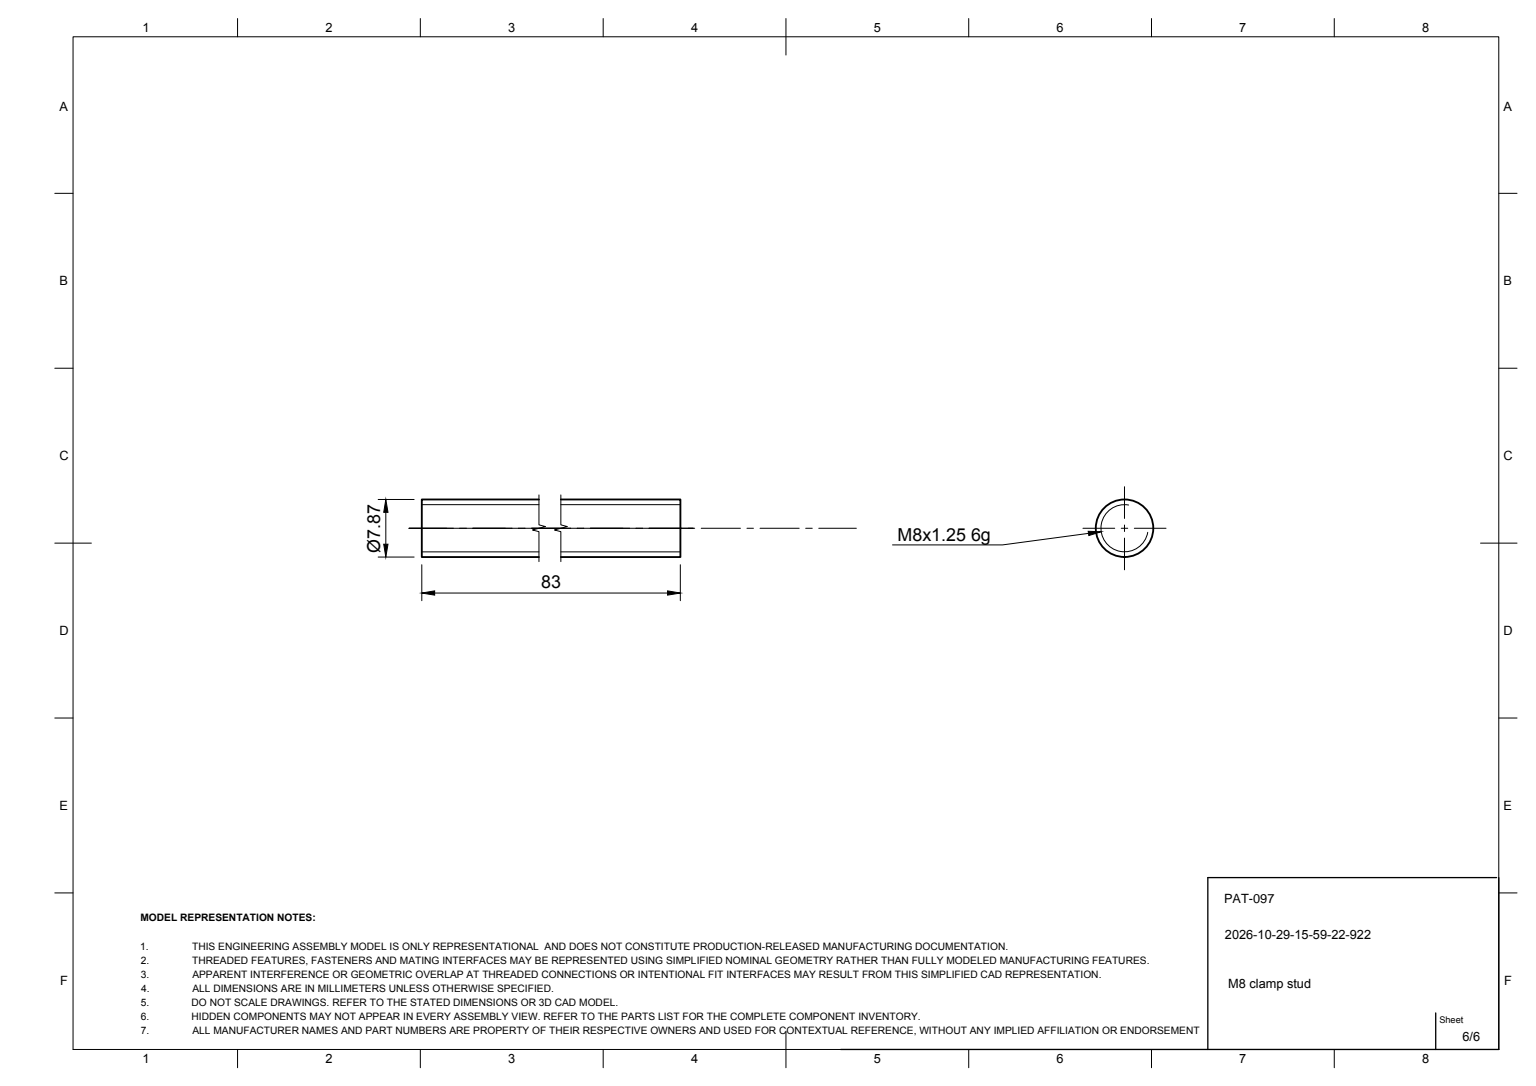
ISO-10303-21;
HEADER;
/* Generated by software containing ST-Developer
 * from STEP Tools, Inc. (www.steptools.com) 
 */

FILE_DESCRIPTION(
/* description */ ('PAT-097'),
/* implementation_level */ '2;1');

FILE_NAME(
/* name */ 'M8 clamp stud.step',
/* time_stamp */ '2026-10-29T15:59:31-07:00',
/* author */ (''),
/* organization */ (''),
/* preprocessor_version */ 'ST-DEVELOPER v20.2',
/* originating_system */ 'Autodesk Translation Framework v15.17.0.0',
/* authorisation */ '');

FILE_SCHEMA (('AUTOMOTIVE_DESIGN { 1 0 10303 214 3 1 1 }'));
ENDSEC;

DATA;
#10=MECHANICAL_DESIGN_GEOMETRIC_PRESENTATION_REPRESENTATION('',(#79),#2768);
#65=SHAPE_REPRESENTATION_RELATIONSHIP('SRR','None',#2803,#72);
#72=ADVANCED_BREP_SHAPE_REPRESENTATION('',(#86),#2765);
#79=STYLED_ITEM('',(#2918),#86);
#86=MANIFOLD_SOLID_BREP('Body1',#1600);
#112=CYLINDRICAL_SURFACE('',#1798,0.3933);
#210=CIRCLE('',#1799,0.3933);
#211=CIRCLE('',#1800,0.3933);
#285=FACE_OUTER_BOUND('',#412,.T.);
#286=FACE_OUTER_BOUND('',#413,.T.);
#287=FACE_OUTER_BOUND('',#414,.T.);
#412=EDGE_LOOP('',(#1391,#1392,#1393,#1394));
#413=EDGE_LOOP('',(#1395));
#414=EDGE_LOOP('',(#1396));
#559=LINE('',#2646,#696);
#696=VECTOR('',#2200,0.4);
#822=VERTEX_POINT('',#2643);
#823=VERTEX_POINT('',#2645);
#1015=EDGE_CURVE('',#822,#822,#210,.F.);
#1016=EDGE_CURVE('',#822,#823,#559,.T.);
#1017=EDGE_CURVE('',#823,#823,#211,.F.);
#1391=ORIENTED_EDGE('',*,*,#1015,.F.);
#1392=ORIENTED_EDGE('',*,*,#1016,.T.);
#1393=ORIENTED_EDGE('',*,*,#1017,.T.);
#1394=ORIENTED_EDGE('',*,*,#1016,.F.);
#1395=ORIENTED_EDGE('',*,*,#1015,.T.);
#1396=ORIENTED_EDGE('',*,*,#1017,.F.);
#1501=PLANE('',#1801);
#1502=PLANE('',#1802);
#1578=ADVANCED_FACE('',(#285),#112,.T.);
#1579=ADVANCED_FACE('',(#286),#1501,.T.);
#1580=ADVANCED_FACE('',(#287),#1502,.F.);
#1600=CLOSED_SHELL('',(#1578,#1579,#1580));
#1797=AXIS2_PLACEMENT_3D('',#2641,#2194,#2195);
#1798=AXIS2_PLACEMENT_3D('',#2642,#2196,#2197);
#1799=AXIS2_PLACEMENT_3D('',#2644,#2198,#2199);
#1800=AXIS2_PLACEMENT_3D('',#2647,#2201,#2202);
#1801=AXIS2_PLACEMENT_3D('',#2648,#2203,#2204);
#1802=AXIS2_PLACEMENT_3D('',#2649,#2205,#2206);
#2194=DIRECTION('axis',(0.,0.,1.));
#2195=DIRECTION('refdir',(1.,0.,0.));
#2196=DIRECTION('center_axis',(0.,0.,1.));
#2197=DIRECTION('ref_axis',(1.,0.,0.));
#2198=DIRECTION('center_axis',(0.,0.,-1.));
#2199=DIRECTION('ref_axis',(1.,0.,0.));
#2200=DIRECTION('',(0.,0.,-1.));
#2201=DIRECTION('center_axis',(0.,0.,-1.));
#2202=DIRECTION('ref_axis',(1.,0.,0.));
#2203=DIRECTION('center_axis',(0.,0.,1.));
#2204=DIRECTION('ref_axis',(1.,0.,0.));
#2205=DIRECTION('center_axis',(0.,0.,1.));
#2206=DIRECTION('ref_axis',(1.,0.,0.));
#2641=CARTESIAN_POINT('',(0.,0.,0.));
#2642=CARTESIAN_POINT('Origin',(10.,-4.,0.));
#2643=CARTESIAN_POINT('',(9.6067,-4.,8.3));
#2644=CARTESIAN_POINT('Origin',(10.,-4.,8.3));
#2645=CARTESIAN_POINT('',(9.6067,-4.,0.));
#2646=CARTESIAN_POINT('',(9.6067,-4.,0.));
#2647=CARTESIAN_POINT('Origin',(10.,-4.,0.));
#2648=CARTESIAN_POINT('Origin',(10.,-4.,8.3));
#2649=CARTESIAN_POINT('Origin',(10.,-4.,0.));
#2756=UNCERTAINTY_MEASURE_WITH_UNIT(LENGTH_MEASURE(0.001),#2769,
'DISTANCE_ACCURACY_VALUE',
'Maximum model space distance between geometric entities at asserted c
onnectivities');
#2759=UNCERTAINTY_MEASURE_WITH_UNIT(LENGTH_MEASURE(0.001),#2769,
'DISTANCE_ACCURACY_VALUE',
'Maximum model space distance between geometric entities at asserted c
onnectivities');
#2765=(
GEOMETRIC_REPRESENTATION_CONTEXT(3)
GLOBAL_UNCERTAINTY_ASSIGNED_CONTEXT((#2756))
GLOBAL_UNIT_ASSIGNED_CONTEXT((#2769,#2771,#2772))
REPRESENTATION_CONTEXT('','3D')
);
#2768=(
GEOMETRIC_REPRESENTATION_CONTEXT(3)
GLOBAL_UNCERTAINTY_ASSIGNED_CONTEXT((#2759))
GLOBAL_UNIT_ASSIGNED_CONTEXT((#2769,#2771,#2772))
REPRESENTATION_CONTEXT('','3D')
);
#2769=(
LENGTH_UNIT()
NAMED_UNIT(*)
SI_UNIT(.CENTI.,.METRE.)
);
#2771=(
NAMED_UNIT(*)
PLANE_ANGLE_UNIT()
SI_UNIT($,.RADIAN.)
);
#2772=(
NAMED_UNIT(*)
SI_UNIT($,.STERADIAN.)
SOLID_ANGLE_UNIT()
);
#2778=SHAPE_DEFINITION_REPRESENTATION(#2786,#2803);
#2786=PRODUCT_DEFINITION_SHAPE('',$,#2812);
#2803=SHAPE_REPRESENTATION('',(#1797),#2765);
#2806=PRODUCT_DEFINITION_CONTEXT('part definition',#2832,'design');
#2812=PRODUCT_DEFINITION('M8 clamp stud','M8 clamp stud',#2820,
#2806);
#2820=PRODUCT_DEFINITION_FORMATION('',$,#2839);
#2832=APPLICATION_CONTEXT(
'Core Data for Automotive Mechanical Design Process');
#2833=PRODUCT_CONTEXT('part definition',#2832,'mechanical');
#2839=PRODUCT('M8 clamp stud','M8 clamp stud',
'M8 clamp stud',(#2833));
#2912=COLOUR_RGB('Black',0.12,0.14,0.17);
#2913=FILL_AREA_STYLE_COLOUR('',#2912);
#2914=FILL_AREA_STYLE('',(#2913));
#2915=SURFACE_STYLE_FILL_AREA(#2914);
#2916=SURFACE_SIDE_STYLE('',(#2915));
#2917=SURFACE_STYLE_USAGE(.BOTH.,#2916);
#2918=PRESENTATION_STYLE_ASSIGNMENT((#2917));
ENDSEC;
END-ISO-10303-21;
